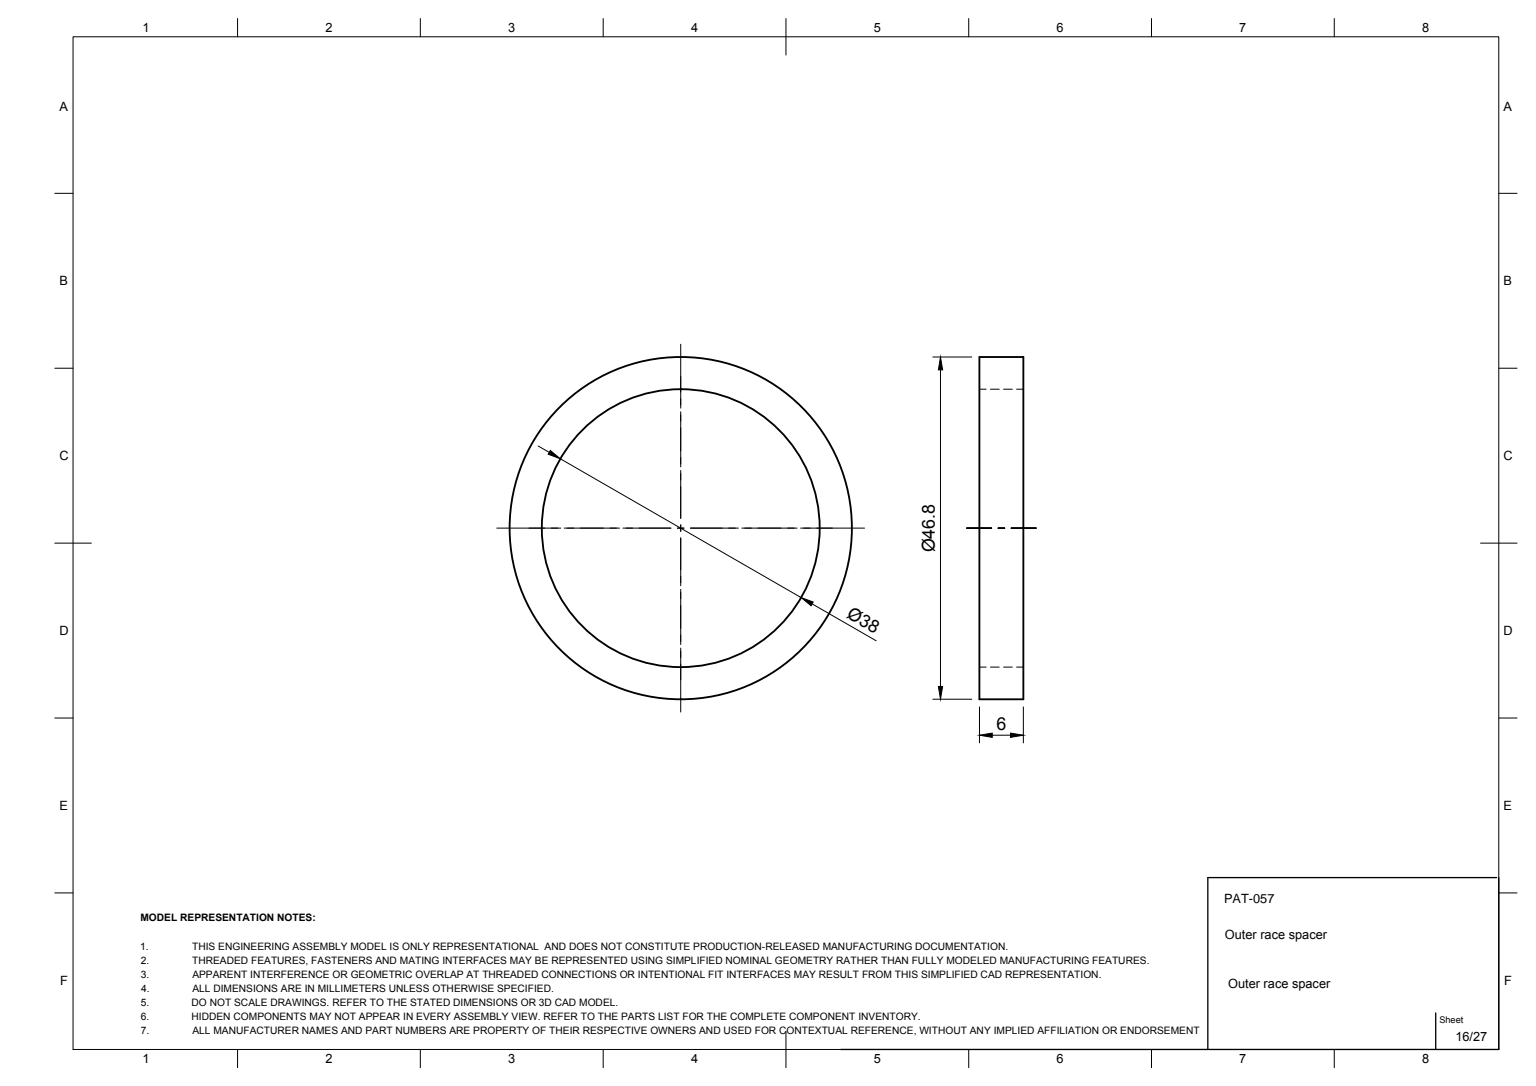
ISO-10303-21;
HEADER;
/* Generated by software containing ST-Developer
 * from STEP Tools, Inc. (www.steptools.com) 
 */

FILE_DESCRIPTION(
/* description */ ('Bearing-mounted hook block'),
/* implementation_level */ '2;1');

FILE_NAME(
/* name */ 'Outer race spacer.step',
/* time_stamp */ '2026-10-28T22:30:11-07:00',
/* author */ (''),
/* organization */ (''),
/* preprocessor_version */ 'ST-DEVELOPER v20.2',
/* originating_system */ 'Autodesk Translation Framework v15.17.0.0',
/* authorisation */ '');

FILE_SCHEMA (('AUTOMOTIVE_DESIGN { 1 0 10303 214 3 1 1 }'));
ENDSEC;

DATA;
#10=MECHANICAL_DESIGN_GEOMETRIC_PRESENTATION_REPRESENTATION('',(#336),#7609);
#288=SHAPE_REPRESENTATION_RELATIONSHIP('SRR','None',#7736,#312);
#312=ADVANCED_BREP_SHAPE_REPRESENTATION('',(#366),#7596);
#336=STYLED_ITEM('',(#7931),#366);
#366=MANIFOLD_SOLID_BREP('Body1',#3934);
#523=LINE('',#6688,#753);
#524=LINE('',#6694,#754);
#753=VECTOR('',#5452,1.9);
#754=VECTOR('',#5459,2.34);
#890=CYLINDRICAL_SURFACE('',#4495,1.9);
#891=CYLINDRICAL_SURFACE('',#4498,2.34);
#972=FACE_BOUND('',#1417,.T.);
#973=FACE_BOUND('',#1419,.T.);
#1127=FACE_OUTER_BOUND('',#1414,.T.);
#1128=FACE_OUTER_BOUND('',#1415,.T.);
#1129=FACE_OUTER_BOUND('',#1416,.T.);
#1130=FACE_OUTER_BOUND('',#1418,.T.);
#1414=EDGE_LOOP('',(#3112,#3113,#3114,#3115));
#1415=EDGE_LOOP('',(#3116,#3117,#3118,#3119));
#1416=EDGE_LOOP('',(#3120));
#1417=EDGE_LOOP('',(#3121));
#1418=EDGE_LOOP('',(#3122));
#1419=EDGE_LOOP('',(#3123));
#1663=CIRCLE('',#4496,1.9);
#1664=CIRCLE('',#4497,1.9);
#1665=CIRCLE('',#4499,2.34);
#1666=CIRCLE('',#4500,2.34);
#1948=VERTEX_POINT('',#6685);
#1949=VERTEX_POINT('',#6687);
#1950=VERTEX_POINT('',#6691);
#1951=VERTEX_POINT('',#6693);
#2366=EDGE_CURVE('',#1948,#1948,#1663,.T.);
#2367=EDGE_CURVE('',#1948,#1949,#523,.T.);
#2368=EDGE_CURVE('',#1949,#1949,#1664,.T.);
#2369=EDGE_CURVE('',#1950,#1950,#1665,.T.);
#2370=EDGE_CURVE('',#1950,#1951,#524,.T.);
#2371=EDGE_CURVE('',#1951,#1951,#1666,.T.);
#3112=ORIENTED_EDGE('',*,*,#2366,.F.);
#3113=ORIENTED_EDGE('',*,*,#2367,.T.);
#3114=ORIENTED_EDGE('',*,*,#2368,.T.);
#3115=ORIENTED_EDGE('',*,*,#2367,.F.);
#3116=ORIENTED_EDGE('',*,*,#2369,.F.);
#3117=ORIENTED_EDGE('',*,*,#2370,.T.);
#3118=ORIENTED_EDGE('',*,*,#2371,.T.);
#3119=ORIENTED_EDGE('',*,*,#2370,.F.);
#3120=ORIENTED_EDGE('',*,*,#2369,.T.);
#3121=ORIENTED_EDGE('',*,*,#2366,.T.);
#3122=ORIENTED_EDGE('',*,*,#2371,.F.);
#3123=ORIENTED_EDGE('',*,*,#2368,.F.);
#3629=PLANE('',#4501);
#3630=PLANE('',#4502);
#3809=ADVANCED_FACE('',(#1127),#890,.F.);
#3810=ADVANCED_FACE('',(#1128),#891,.T.);
#3811=ADVANCED_FACE('',(#1129,#972),#3629,.T.);
#3812=ADVANCED_FACE('',(#1130,#973),#3630,.F.);
#3934=CLOSED_SHELL('',(#3809,#3810,#3811,#3812));
#4494=AXIS2_PLACEMENT_3D('',#6683,#5446,#5447);
#4495=AXIS2_PLACEMENT_3D('',#6684,#5448,#5449);
#4496=AXIS2_PLACEMENT_3D('',#6686,#5450,#5451);
#4497=AXIS2_PLACEMENT_3D('',#6689,#5453,#5454);
#4498=AXIS2_PLACEMENT_3D('',#6690,#5455,#5456);
#4499=AXIS2_PLACEMENT_3D('',#6692,#5457,#5458);
#4500=AXIS2_PLACEMENT_3D('',#6695,#5460,#5461);
#4501=AXIS2_PLACEMENT_3D('',#6696,#5462,#5463);
#4502=AXIS2_PLACEMENT_3D('',#6697,#5464,#5465);
#5446=DIRECTION('axis',(0.,0.,1.));
#5447=DIRECTION('refdir',(1.,0.,0.));
#5448=DIRECTION('center_axis',(0.,1.,0.));
#5449=DIRECTION('ref_axis',(1.,0.,0.));
#5450=DIRECTION('center_axis',(0.,-1.,0.));
#5451=DIRECTION('ref_axis',(1.,0.,0.));
#5452=DIRECTION('',(0.,-1.,0.));
#5453=DIRECTION('center_axis',(0.,-1.,0.));
#5454=DIRECTION('ref_axis',(1.,0.,0.));
#5455=DIRECTION('center_axis',(0.,1.,0.));
#5456=DIRECTION('ref_axis',(1.,0.,0.));
#5457=DIRECTION('center_axis',(0.,1.,0.));
#5458=DIRECTION('ref_axis',(1.,0.,0.));
#5459=DIRECTION('',(0.,-1.,0.));
#5460=DIRECTION('center_axis',(0.,1.,0.));
#5461=DIRECTION('ref_axis',(1.,0.,0.));
#5462=DIRECTION('center_axis',(0.,1.,0.));
#5463=DIRECTION('ref_axis',(1.,0.,0.));
#5464=DIRECTION('center_axis',(0.,1.,0.));
#5465=DIRECTION('ref_axis',(1.,0.,0.));
#6683=CARTESIAN_POINT('',(0.,0.,0.));
#6684=CARTESIAN_POINT('Origin',(0.,-0.3,12.));
#6685=CARTESIAN_POINT('',(-1.9,0.3,12.));
#6686=CARTESIAN_POINT('Origin',(0.,0.3,12.));
#6687=CARTESIAN_POINT('',(-1.9,-0.3,12.));
#6688=CARTESIAN_POINT('',(-1.9,-0.3,12.));
#6689=CARTESIAN_POINT('Origin',(0.,-0.3,12.));
#6690=CARTESIAN_POINT('Origin',(0.,-0.3,12.));
#6691=CARTESIAN_POINT('',(-2.34,0.3,12.));
#6692=CARTESIAN_POINT('Origin',(0.,0.3,12.));
#6693=CARTESIAN_POINT('',(-2.34,-0.3,12.));
#6694=CARTESIAN_POINT('',(-2.34,-0.3,12.));
#6695=CARTESIAN_POINT('Origin',(0.,-0.3,12.));
#6696=CARTESIAN_POINT('Origin',(0.,0.3,12.));
#6697=CARTESIAN_POINT('Origin',(0.,-0.3,12.));
#7566=UNCERTAINTY_MEASURE_WITH_UNIT(LENGTH_MEASURE(0.001),#7610,
'DISTANCE_ACCURACY_VALUE',
'Maximum model space distance between geometric entities at asserted c
onnectivities');
#7579=UNCERTAINTY_MEASURE_WITH_UNIT(LENGTH_MEASURE(0.001),#7610,
'DISTANCE_ACCURACY_VALUE',
'Maximum model space distance between geometric entities at asserted c
onnectivities');
#7596=(
GEOMETRIC_REPRESENTATION_CONTEXT(3)
GLOBAL_UNCERTAINTY_ASSIGNED_CONTEXT((#7566))
GLOBAL_UNIT_ASSIGNED_CONTEXT((#7610,#7612,#7613))
REPRESENTATION_CONTEXT('','3D')
);
#7609=(
GEOMETRIC_REPRESENTATION_CONTEXT(3)
GLOBAL_UNCERTAINTY_ASSIGNED_CONTEXT((#7579))
GLOBAL_UNIT_ASSIGNED_CONTEXT((#7610,#7612,#7613))
REPRESENTATION_CONTEXT('','3D')
);
#7610=(
LENGTH_UNIT()
NAMED_UNIT(*)
SI_UNIT(.CENTI.,.METRE.)
);
#7612=(
NAMED_UNIT(*)
PLANE_ANGLE_UNIT()
SI_UNIT($,.RADIAN.)
);
#7613=(
NAMED_UNIT(*)
SI_UNIT($,.STERADIAN.)
SOLID_ANGLE_UNIT()
);
#7630=SHAPE_DEFINITION_REPRESENTATION(#7682,#7736);
#7682=PRODUCT_DEFINITION_SHAPE('',$,#7766);
#7736=SHAPE_REPRESENTATION('',(#4494),#7596);
#7749=PRODUCT_DEFINITION_CONTEXT('part definition',#7838,'design');
#7766=PRODUCT_DEFINITION('Outer race spacer','Outer race spacer',#7795,
#7749);
#7795=PRODUCT_DEFINITION_FORMATION('',$,#7856);
#7838=APPLICATION_CONTEXT(
'Core Data for Automotive Mechanical Design Process');
#7839=PRODUCT_CONTEXT('part definition',#7838,'mechanical');
#7856=PRODUCT('Outer race spacer','Outer race spacer',
'Outer race spacer',(#7839));
#7925=COLOUR_RGB('Grey',0.48,0.52,0.57);
#7926=FILL_AREA_STYLE_COLOUR('',#7925);
#7927=FILL_AREA_STYLE('',(#7926));
#7928=SURFACE_STYLE_FILL_AREA(#7927);
#7929=SURFACE_SIDE_STYLE('',(#7928));
#7930=SURFACE_STYLE_USAGE(.BOTH.,#7929);
#7931=PRESENTATION_STYLE_ASSIGNMENT((#7930));
ENDSEC;
END-ISO-10303-21;
